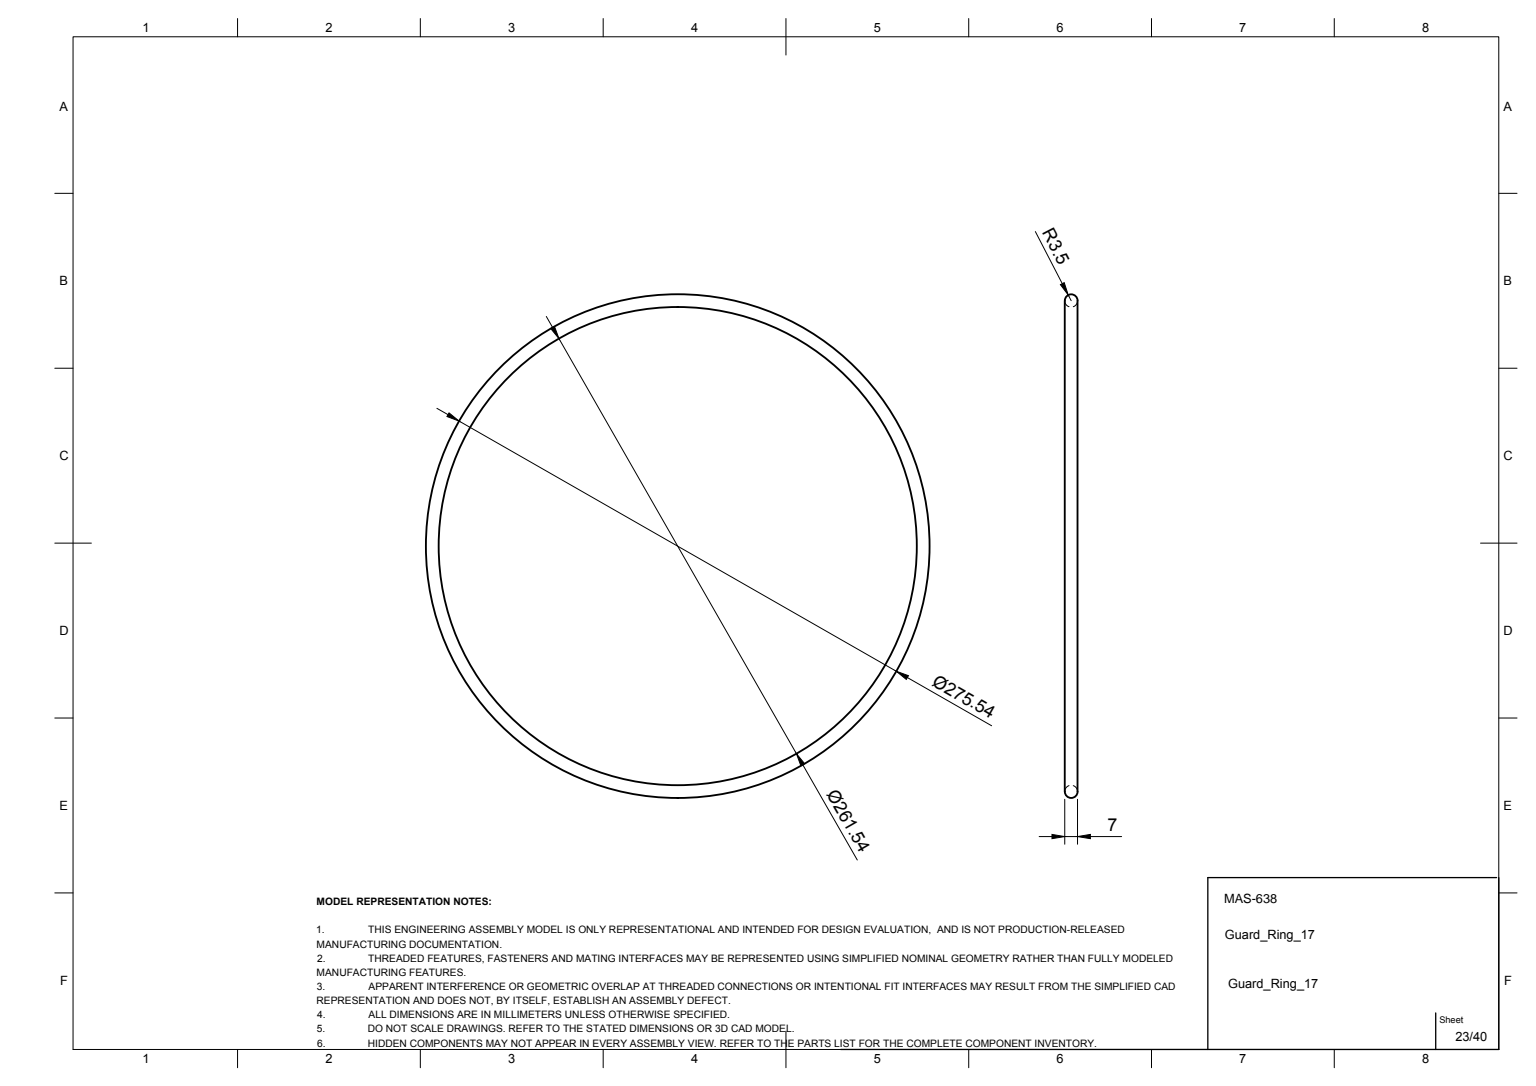
ISO-10303-21;
HEADER;
FILE_DESCRIPTION((''),'2;1');
FILE_NAME('Guard_Ring_17.step','2026-10-09T12:00:21-07:00',(''),(''),'','','');
FILE_SCHEMA (('AUTOMOTIVE_DESIGN { 1 0 10303 214 3 1 1 }'));
ENDSEC;
DATA;
#10=MECHANICAL_DESIGN_GEOMETRIC_PRESENTATION_REPRESENTATION('',(#422),#10334);
#350=SHAPE_REPRESENTATION_RELATIONSHIP('SRR','None',#10466,#382) ;
#382=ADVANCED_BREP_SHAPE_REPRESENTATION('',(#454),#10318) ;
#422=STYLED_ITEM('',(#10631),#454) ;
#454=MANIFOLD_SOLID_BREP('Body1',#3576) ;
#875=FACE_OUTER_BOUND('',#1075,.T.) ;
#1075=EDGE_LOOP('',(#2413,#2414,#2415,#2416)) ;
#1308=CIRCLE('',#4039,0.349999999999999) ;
#1309=CIRCLE('',#4040,13.0768144613668) ;
#1529=VERTEX_POINT('',#5733) ;
#1863=EDGE_CURVE('',#1529,#1529,#1308,.T.) ;
#1864=EDGE_CURVE('',#1529,#1529,#1309,.T.) ;
#2413=ORIENTED_EDGE('',*,*,#1863,.F.) ;
#2414=ORIENTED_EDGE('',*,*,#1864,.T.) ;
#2415=ORIENTED_EDGE('',*,*,#1863,.T.) ;
#2416=ORIENTED_EDGE('',*,*,#1864,.F.) ;
#3321=TOROIDAL_SURFACE('',#4038,13.4268144613668,0.349999999999999) ;
#3383=ADVANCED_FACE('',(#875),#3321,.T.) ;
#3576=CLOSED_SHELL('',(#3383)) ;
#4037=AXIS2_PLACEMENT_3D('',#5731,#4635,#4636) ;
#4038=AXIS2_PLACEMENT_3D('',#5732,#4637,#4638) ;
#4039=AXIS2_PLACEMENT_3D('',#5734,#4639,#4640) ;
#4040=AXIS2_PLACEMENT_3D('',#5735,#4641,#4642) ;
#4635=DIRECTION('axis',(0.,0.,1.)) ;
#4636=DIRECTION('refdir',(1.,0.,0.)) ;
#4637=DIRECTION('center_axis',(-6.42891162084177E-17,-1.,-1.01883556321148E-16)) ;
#4638=DIRECTION('ref_axis',(1.,0.,0.)) ;
#4639=DIRECTION('center_axis',(0.,1.01883556321148E-16,-1.)) ;
#4640=DIRECTION('ref_axis',(-1.,0.,0.)) ;
#4641=DIRECTION('center_axis',(6.42891162084177E-17,1.,1.01883556321148E-16)) ;
#4642=DIRECTION('ref_axis',(1.,-6.42891162084177E-17,-6.55000379205715E-33)) ;
#5731=CARTESIAN_POINT('',(0.,0.,0.)) ;
#5732=CARTESIAN_POINT('Origin',(23.47768801576,65.9831179463143,68.2224337400009)) ;
#5733=CARTESIAN_POINT('',(10.4008735543932,65.9831179463143,68.2224337400009)) ;
#5734=CARTESIAN_POINT('Origin',(10.0508735543932,65.9831179463143,68.2224337400009)) ;
#5735=CARTESIAN_POINT('Origin',(23.47768801576,65.9831179463143,68.2224337400009)) ;
#10281=UNCERTAINTY_MEASURE_WITH_UNIT(LENGTH_MEASURE(0.001),#10335,
'DISTANCE_ACCURACY_VALUE',
'Maximum model space distance between geometric entities at asserted c
onnectivities') ;
#10297=UNCERTAINTY_MEASURE_WITH_UNIT(LENGTH_MEASURE(0.001),#10335,
'DISTANCE_ACCURACY_VALUE',
'Maximum model space distance between geometric entities at asserted c
onnectivities') ;
#10318=(
GEOMETRIC_REPRESENTATION_CONTEXT(3)
GLOBAL_UNCERTAINTY_ASSIGNED_CONTEXT((#10281))
GLOBAL_UNIT_ASSIGNED_CONTEXT((#10335,#10337,#10338))
REPRESENTATION_CONTEXT('','3D')
) ;
#10334=(
GEOMETRIC_REPRESENTATION_CONTEXT(3)
GLOBAL_UNCERTAINTY_ASSIGNED_CONTEXT((#10297))
GLOBAL_UNIT_ASSIGNED_CONTEXT((#10335,#10337,#10338))
REPRESENTATION_CONTEXT('','3D')
) ;
#10335=(
LENGTH_UNIT()
NAMED_UNIT(*)
SI_UNIT(.CENTI.,.METRE.)
) ;
#10337=(
NAMED_UNIT(*)
PLANE_ANGLE_UNIT()
SI_UNIT($,.RADIAN.)
) ;
#10338=(
NAMED_UNIT(*)
SI_UNIT($,.STERADIAN.)
SOLID_ANGLE_UNIT()
) ;
#10359=SHAPE_DEFINITION_REPRESENTATION(#10395,#10466) ;
#10395=PRODUCT_DEFINITION_SHAPE('',$,#10503) ;
#10466=SHAPE_REPRESENTATION('',(#4037),#10318) ;
#10482=PRODUCT_DEFINITION_CONTEXT('part definition',#10592,'design') ;
#10503=PRODUCT_DEFINITION('Guard_Ring_17','Guard_Ring_17',#10539,#10482) ;
#10539=PRODUCT_DEFINITION_FORMATION('',$,#10614) ;
#10592=APPLICATION_CONTEXT(
'Core Data for Automotive Mechanical Design Process') ;
#10593=PRODUCT_CONTEXT('part definition',#10592,'mechanical') ;
#10614=PRODUCT('Guard_Ring_17','Guard_Ring_17',$,(#10593)) ;
#10631=PRESENTATION_STYLE_ASSIGNMENT((#10635)) ;
#10635=SURFACE_STYLE_USAGE(.BOTH.,#10639) ;
#10639=SURFACE_SIDE_STYLE('',(#10643)) ;
#10643=SURFACE_STYLE_FILL_AREA(#10647) ;
#10647=FILL_AREA_STYLE('Opaque(25,25,25)',(#10651)) ;
#10651=FILL_AREA_STYLE_COLOUR('Opaque(25,25,25)',#10655) ;
#10655=COLOUR_RGB('Opaque(25,25,25)', 0.09019608, 0.27058824, 0.51372549) ;
ENDSEC;
END-ISO-10303-21;
